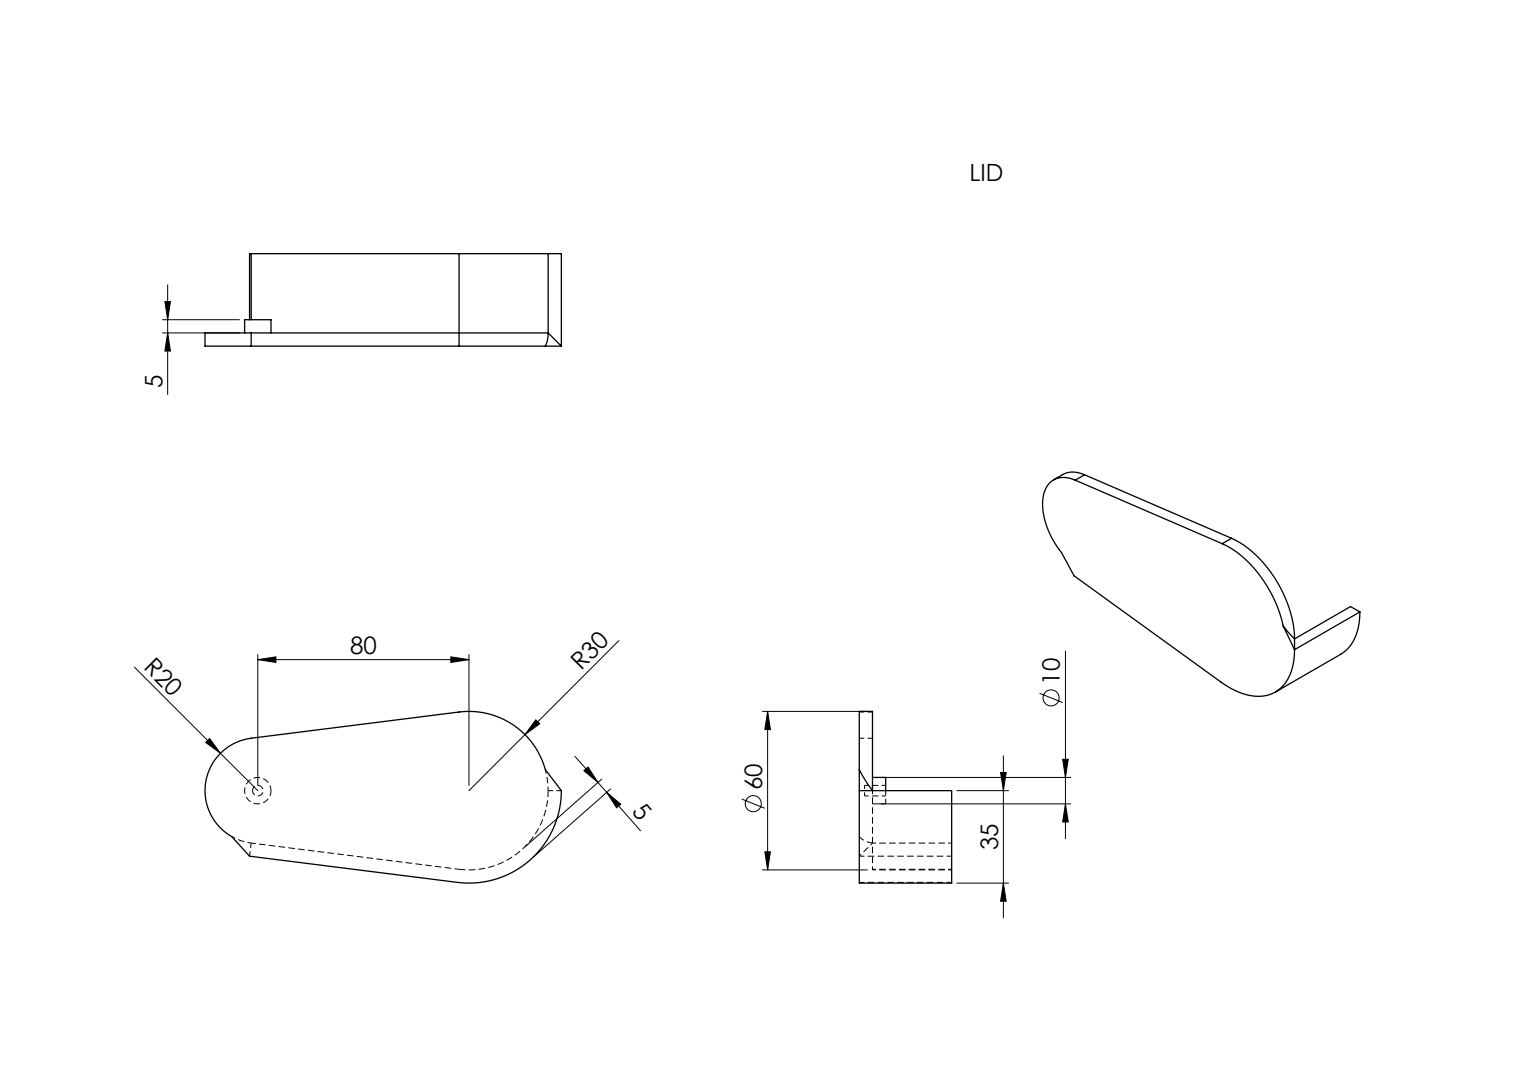
ISO-10303-21;
HEADER;
FILE_DESCRIPTION (('STEP AP214'),
    '1' );
FILE_NAME ('lid.step',
    '2026-10-24T08:20:21',
    ( '' ),
    ( '' ),
    'SwSTEP 2.0',
    'SolidWorks 2026',
    '' );
FILE_SCHEMA (( 'AUTOMOTIVE_DESIGN' ));
ENDSEC;

DATA;
#5=ORIENTED_EDGE ( 'NONE', *, *, #1076, .T. ) ;
#24=VECTOR ( 'NONE', #1964, 1000.000000000000000 ) ;
#27=CARTESIAN_POINT ( 'NONE',  ( -85.00000000000000000, 6.123233995736770227E-16, 0.000000000000000000 ) ) ;
#30=ORIENTED_EDGE ( 'NONE', *, *, #1022, .T. ) ;
#33=CIRCLE ( 'NONE', #906, 20.00000000000000355 ) ;
#34=EDGE_CURVE ( 'NONE', #3645, #1107, #2841, .T. ) ;
#40=COLOUR_RGB ( '',0.8941176470588234615, 0.8941176470588234615, 0.8941176470588234615 ) ;
#45=( LENGTH_UNIT ( ) NAMED_UNIT ( * ) SI_UNIT ( .MILLI., .METRE. ) );
#47=PLANE ( 'NONE',  #2813 ) ;
#66=CARTESIAN_POINT ( 'NONE',  ( -80.00000000000000000, 0.000000000000000000, -5.000000000000000000 ) ) ;
#68=CARTESIAN_POINT ( 'NONE',  ( -80.00000000000000000, 0.000000000000000000, 0.000000000000000000 ) ) ;
#73=CARTESIAN_POINT ( 'NONE',  ( -80.00000000000000000, 0.000000000000000000, -5.000000000000000000 ) ) ;
#86=ORIENTED_EDGE ( 'NONE', *, *, #1066, .F. ) ;
#92=CARTESIAN_POINT ( 'NONE',  ( 28.92857142857272379, 7.945926950454914817, 5.000000000000000000 ) ) ;
#100=EDGE_CURVE ( 'NONE', #2912, #2597, #2303, .T. ) ;
#119=DIRECTION ( 'NONE',  ( -0.000000000000000000, 0.000000000000000000, 1.000000000000000000 ) ) ;
#121=PLANE ( 'NONE',  #644 ) ;
#131=VECTOR ( 'NONE', #1399, 1000.000000000000000 ) ;
#132=AXIS2_PLACEMENT_3D ( 'NONE', #1292, #3708, #687 ) ;
#135=EDGE_LOOP ( 'NONE', ( #399, #815 ) ) ;
#138=CARTESIAN_POINT ( 'NONE',  ( -83.12500000000000000, -24.80391854123052653, 5.000000000000000000 ) ) ;
#145=EDGE_CURVE ( 'NONE', #3052, #3455, #33, .T. ) ;
#151=EDGE_CURVE ( 'NONE', #2912, #447, #915, .T. ) ;
#155=FACE_OUTER_BOUND ( 'NONE', #841, .T. ) ;
#157=EDGE_CURVE ( 'NONE', #2149, #2587, #627, .T. ) ;
#160=ORIENTED_EDGE ( 'NONE', *, *, #2560, .F. ) ;
#176=CARTESIAN_POINT ( 'NONE',  ( 0.000000000000000000, 0.000000000000000000, -30.00000000000000000 ) ) ;
#182=DIRECTION ( 'NONE',  ( -0.000000000000000000, 0.000000000000000000, 1.000000000000000000 ) ) ;
#183=ORIENTED_EDGE ( 'NONE', *, *, #151, .F. ) ;
#184=LINE ( 'NONE', #240, #851 ) ;
#187=CARTESIAN_POINT ( 'NONE',  ( -82.50000000000000000, -19.84313483298442904, 0.000000000000000000 ) ) ;
#194=FACE_OUTER_BOUND ( 'NONE', #457, .T. ) ;
#198=( GEOMETRIC_REPRESENTATION_CONTEXT ( 3 ) GLOBAL_UNCERTAINTY_ASSIGNED_CONTEXT ( ( #1403 ) ) GLOBAL_UNIT_ASSIGNED_CONTEXT ( ( #953, #339, #637 ) ) REPRESENTATION_CONTEXT ( 'NONE', 'WORKASPACE' ) );
#202=CARTESIAN_POINT ( 'NONE',  ( 28.92857142857272379, 7.945926950454914817, 5.000000000000000000 ) ) ;
#210=DIRECTION ( 'NONE',  ( 1.000000000000000000, 0.000000000000000000, 0.000000000000000000 ) ) ;
#217=CARTESIAN_POINT ( 'NONE',  ( -85.13135963406439544, -19.37413418176162594, 2.144658748104447454 ) ) ;
#222=FACE_OUTER_BOUND ( 'NONE', #2249, .T. ) ;
#228=CARTESIAN_POINT ( 'NONE',  ( -80.00000000000000000, 0.000000000000000000, -5.000000000000000000 ) ) ;
#230=EDGE_LOOP ( 'NONE', ( #423, #458, #2940, #857 ) ) ;
#236=B_SPLINE_CURVE_WITH_KNOTS ( 'NONE', 3,
 ( #2282, #3465, #1982, #3172 ),
 .UNSPECIFIED., .F., .F.,
 ( 4, 4 ),
 ( 0.000000000000000000, 1.000000000000000000 ),
 .UNSPECIFIED. ) ;
#238=PLANE ( 'NONE',  #1875 ) ;
#240=CARTESIAN_POINT ( 'NONE',  ( -4.374999999999999112, -34.72548595772274638, -30.00000000000000000 ) ) ;
#248=CARTESIAN_POINT ( 'NONE',  ( -4.375000000000000888, -34.72548595772274638, 5.000000000000000000 ) ) ;
#250=ADVANCED_FACE ( 'NONE', ( #2060 ), #299, .T. ) ;
#254=ORIENTED_EDGE ( 'NONE', *, *, #3594, .F. ) ;
#269=B_SPLINE_CURVE_WITH_KNOTS ( 'NONE', 3,
 ( #2225, #1680, #3784, #502 ),
 .UNSPECIFIED., .F., .F.,
 ( 4, 4 ),
 ( 0.000000000000000000, 1.000000000000000000 ),
 .UNSPECIFIED. ) ;
#272=VERTEX_POINT ( 'NONE', #897 ) ;
#288=B_SPLINE_CURVE_WITH_KNOTS ( 'NONE', 3,
 ( #1129, #864, #2961, #3833 ),
 .UNSPECIFIED., .F., .F.,
 ( 4, 4 ),
 ( 0.000000000000000000, 1.000000000000000000 ),
 .UNSPECIFIED. ) ;
#292=DIRECTION ( 'NONE',  ( 0.000000000000000000, 0.000000000000000000, 1.000000000000000000 ) ) ;
#297=ORIENTED_EDGE ( 'NONE', *, *, #1259, .F. ) ;
#299=CYLINDRICAL_SURFACE ( 'NONE', #1463, 20.00000000000000355 ) ;
#305=DIRECTION ( 'NONE',  ( -0.9921567416492215186, 0.1250000000000000833, 0.000000000000000000 ) ) ;
#318=VECTOR ( 'NONE', #1119, 999.9999999999998863 ) ;
#323=VECTOR ( 'NONE', #1438, 1000.000000000000114 ) ;
#327=AXIS2_PLACEMENT_3D ( 'NONE', #856, #2331, #1108 ) ;
#329=PLANE ( 'NONE',  #132 ) ;
#339=( NAMED_UNIT ( * ) PLANE_ANGLE_UNIT ( ) SI_UNIT ( $, .RADIAN. ) );
#340=MECHANICAL_DESIGN_GEOMETRIC_PRESENTATION_REPRESENTATION('',(#468),#3515);
#343=PRODUCT ( 'lid', 'lid', '', ( #1165 ) ) ;
#356=LINE ( 'NONE', #1470, #3071 ) ;
#371=CARTESIAN_POINT ( 'NONE',  ( 34.99999999999999289, 0.000000000000000000, -30.00000000000000000 ) ) ;
#382=EDGE_CURVE ( 'NONE', #2840, #3645, #603, .T. ) ;
#388=EDGE_CURVE ( 'NONE', #973, #1542, #2135, .T. ) ;
#392=CARTESIAN_POINT ( 'NONE',  ( 30.00000000000000000, 0.000000000000000000, -15.00000000000000000 ) ) ;
#399=ORIENTED_EDGE ( 'NONE', *, *, #1610, .T. ) ;
#403=VECTOR ( 'NONE', #2056, 1000.000000000000000 ) ;
#405=DIRECTION ( 'NONE',  ( 0.000000000000000000, 0.000000000000000000, 1.000000000000000000 ) ) ;
#407=FACE_OUTER_BOUND ( 'NONE', #796, .T. ) ;
#414=LINE ( 'NONE', #2795, #24 ) ;
#415=EDGE_LOOP ( 'NONE', ( #3354, #1082 ) ) ;
#422=EDGE_CURVE ( 'NONE', #2840, #2012, #3114, .T. ) ;
#423=ORIENTED_EDGE ( 'NONE', *, *, #3594, .T. ) ;
#430=CARTESIAN_POINT ( 'NONE',  ( 0.000000000000000000, 0.000000000000000000, -30.00000000000000000 ) ) ;
#447=VERTEX_POINT ( 'NONE', #1262 ) ;
#453=EDGE_LOOP ( 'NONE', ( #297, #1815, #2065, #876 ) ) ;
#456=FACE_OUTER_BOUND ( 'NONE', #836, .T. ) ;
#457=EDGE_LOOP ( 'NONE', ( #3256, #3221, #3322, #30 ) ) ;
#458=ORIENTED_EDGE ( 'NONE', *, *, #1532, .F. ) ;
#468=STYLED_ITEM ( 'NONE', ( #939 ), #3116 ) ;
#490=LINE ( 'NONE', #3484, #318 ) ;
#502=CARTESIAN_POINT ( 'NONE',  ( 28.92857142857272379, 7.945926950454914817, 5.000000000000000000 ) ) ;
#503=ORIENTED_EDGE ( 'NONE', *, *, #2320, .F. ) ;
#505=CARTESIAN_POINT ( 'NONE',  ( -82.50000000000000000, -19.84313483298442904, 0.000000000000000000 ) ) ;
#506=EDGE_LOOP ( 'NONE', ( #2013, #1714, #3610, #3275 ) ) ;
#534=DIRECTION ( 'NONE',  ( 0.6221102074731698073, 0.4753501651576230724, -0.6221102074731695852 ) ) ;
#536=CARTESIAN_POINT ( 'NONE',  ( -4.375000000000001776, -34.72548595772274638, -30.00000000000000000 ) ) ;
#537=PRODUCT_DEFINITION ( 'UNKNOWN', '', #3334, #2544 ) ;
#541=DIRECTION ( 'NONE',  ( -0.000000000000000000, -0.000000000000000000, 1.000000000000000000 ) ) ;
#571=ORIENTED_EDGE ( 'NONE', *, *, #2102, .F. ) ;
#577=AXIS2_PLACEMENT_3D ( 'NONE', #710, #3339, #1868 ) ;
#603=LINE ( 'NONE', #2116, #3452 ) ;
#613=ORIENTED_EDGE ( 'NONE', *, *, #1657, .T. ) ;
#627=B_SPLINE_CURVE_WITH_KNOTS ( 'NONE', 3,
 ( #187, #1692, #2876, #2337 ),
 .UNSPECIFIED., .F., .F.,
 ( 4, 4 ),
 ( 0.000000000000000000, 1.000000000000000000 ),
 .UNSPECIFIED. ) ;
#633=ORIENTED_EDGE ( 'NONE', *, *, #1532, .T. ) ;
#637=( NAMED_UNIT ( * ) SI_UNIT ( $, .STERADIAN. ) SOLID_ANGLE_UNIT ( ) );
#642=CARTESIAN_POINT ( 'NONE',  ( 29.64285714285758999, 5.345441766669614125, 3.727272727272256336 ) ) ;
#644=AXIS2_PLACEMENT_3D ( 'NONE', #2215, #2193, #3654 ) ;
#645=AXIS2_PLACEMENT_3D ( 'NONE', #68, #3596, #933 ) ;
#651=ORIENTED_EDGE ( 'NONE', *, *, #3049, .T. ) ;
#658=LINE ( 'NONE', #1244, #2009 ) ;
#663=( NAMED_UNIT ( * ) SI_UNIT ( $, .STERADIAN. ) SOLID_ANGLE_UNIT ( ) );
#664=AXIS2_PLACEMENT_3D ( 'NONE', #2506, #2533, #3696 ) ;
#670=DIRECTION ( 'NONE',  ( -0.1250000000000000555, -0.9921567416492214075, 0.000000000000000000 ) ) ;
#680=( LENGTH_UNIT ( ) NAMED_UNIT ( * ) SI_UNIT ( .MILLI., .METRE. ) );
#687=DIRECTION ( 'NONE',  ( -1.000000000000000000, 0.000000000000000000, -0.000000000000000000 ) ) ;
#700=SHAPE_REPRESENTATION_RELATIONSHIP ( 'NONE' , 'NONE' ,  #2152, #3116 ) ;
#704=AXIS2_PLACEMENT_3D ( 'NONE', #430, #1338, #1604 ) ;
#706=CARTESIAN_POINT ( 'NONE',  ( -3.749999999999998224, -29.76470224947664533, 0.000000000000000000 ) ) ;
#709=ORIENTED_EDGE ( 'NONE', *, *, #3416, .F. ) ;
#710=CARTESIAN_POINT ( 'NONE',  ( -78.00000000000000000, 0.000000000000000000, 3.000000000000000000 ) ) ;
#720=AXIS2_PLACEMENT_3D ( 'NONE', #176, #788, #1721 ) ;
#722=DIRECTION ( 'NONE',  ( 1.000000000000000000, 0.000000000000000000, 0.000000000000000000 ) ) ;
#733=DIRECTION ( 'NONE',  ( -1.000000000000000000, 0.000000000000000000, 0.000000000000000000 ) ) ;
#734=EDGE_CURVE ( 'NONE', #916, #926, #1606, .T. ) ;
#735=DIRECTION ( 'NONE',  ( 1.000000000000000000, 0.000000000000000000, 0.000000000000000000 ) ) ;
#743=CARTESIAN_POINT ( 'NONE',  ( -80.00000000000000000, 0.000000000000000000, -5.000000000000000000 ) ) ;
#752=DIRECTION ( 'NONE',  ( 0.9921567416492214075, 0.1250000000000001388, 0.000000000000000000 ) ) ;
#753=ORIENTED_EDGE ( 'NONE', *, *, #1610, .F. ) ;
#754=CARTESIAN_POINT ( 'NONE',  ( 34.99999999999999289, 0.000000000000000000, 4.999999999999997335 ) ) ;
#756=FACE_OUTER_BOUND ( 'NONE', #3199, .T. ) ;
#763=CIRCLE ( 'NONE', #1018, 34.99999999999999289 ) ;
#765=CIRCLE ( 'NONE', #2944, 2.000000000000001776 ) ;
#773=ORIENTED_EDGE ( 'NONE', *, *, #2847, .T. ) ;
#780=CARTESIAN_POINT ( 'NONE',  ( -82.50000000000000000, 19.84313483298442193, 0.000000000000000000 ) ) ;
#788=DIRECTION ( 'NONE',  ( 0.000000000000000000, 0.000000000000000000, 1.000000000000000000 ) ) ;
#796=EDGE_LOOP ( 'NONE', ( #3689, #2096 ) ) ;
#806=DIRECTION ( 'NONE',  ( -0.9921567416492214075, 0.1250000000000000555, 0.000000000000000000 ) ) ;
#815=ORIENTED_EDGE ( 'NONE', *, *, #2560, .T. ) ;
#819=DIRECTION ( 'NONE',  ( 0.000000000000000000, 0.000000000000000000, 1.000000000000000000 ) ) ;
#820=CARTESIAN_POINT ( 'NONE',  ( 0.000000000000000000, 0.000000000000000000, 0.000000000000000000 ) ) ;
#821=VERTEX_POINT ( 'NONE', #3348 ) ;
#822=VECTOR ( 'NONE', #1593, 999.9999999999998863 ) ;
#828=UNCERTAINTY_MEASURE_WITH_UNIT (LENGTH_MEASURE( 1.000000000000000082E-05 ), #45, 'distance_accuracy_value', 'NONE');
#831=FACE_OUTER_BOUND ( 'NONE', #3651, .T. ) ;
#832=VECTOR ( 'NONE', #405, 1000.000000000000000 ) ;
#836=EDGE_LOOP ( 'NONE', ( #1395, #5, #966, #3713, #3401, #3386 ) ) ;
#837=CARTESIAN_POINT ( 'NONE',  ( -80.00000000000000000, 0.000000000000000000, 5.000000000000000000 ) ) ;
#841=EDGE_LOOP ( 'NONE', ( #254, #990, #1674, #1273, #1658, #1329, #1704 ) ) ;
#845=ADVANCED_FACE ( 'NONE', ( #3670 ), #1013, .T. ) ;
#851=VECTOR ( 'NONE', #3438, 1000.000000000000000 ) ;
#856=CARTESIAN_POINT ( 'NONE',  ( 0.000000000000000000, 0.000000000000000000, 0.000000000000000000 ) ) ;
#857=ORIENTED_EDGE ( 'NONE', *, *, #1052, .T. ) ;
#860=ADVANCED_FACE ( 'NONE', ( #1357 ), #1602, .T. ) ;
#864=CARTESIAN_POINT ( 'NONE',  ( -85.36741282452705093, -22.33760634779116572, 4.999999999999999112 ) ) ;
#868=VERTEX_POINT ( 'NONE', #2547 ) ;
#869=LINE ( 'NONE', #2673, #2691 ) ;
#876=ORIENTED_EDGE ( 'NONE', *, *, #1758, .T. ) ;
#879=ORIENTED_EDGE ( 'NONE', *, *, #3782, .F. ) ;
#882=ORIENTED_EDGE ( 'NONE', *, *, #3649, .T. ) ;
#893=MECHANICAL_DESIGN_GEOMETRIC_PRESENTATION_REPRESENTATION('',(#2124),#198);
#897=CARTESIAN_POINT ( 'NONE',  ( -82.00000000000000000, 0.000000000000000000, 3.000000000000000000 ) ) ;
#906=AXIS2_PLACEMENT_3D ( 'NONE', #837, #3174, #2024 ) ;
#910=VERTEX_POINT ( 'NONE', #1069 ) ;
#913=AXIS2_PLACEMENT_3D ( 'NONE', #1710, #2640, #3753 ) ;
#915=CIRCLE ( 'NONE', #2590, 5.000000000000004441 ) ;
#916=VERTEX_POINT ( 'NONE', #371 ) ;
#926=VERTEX_POINT ( 'NONE', #754 ) ;
#930=EDGE_CURVE ( 'NONE', #1166, #1798, #1457, .T. ) ;
#933=DIRECTION ( 'NONE',  ( 1.000000000000000000, 0.000000000000000000, 0.000000000000000000 ) ) ;
#939=PRESENTATION_STYLE_ASSIGNMENT (( #2140 ) ) ;
#941=CARTESIAN_POINT ( 'NONE',  ( -82.50000000000000000, -19.84313483298442904, -30.00000000000000000 ) ) ;
#951=DIRECTION ( 'NONE',  ( 0.000000000000000000, 0.000000000000000000, 1.000000000000000000 ) ) ;
#953=( LENGTH_UNIT ( ) NAMED_UNIT ( * ) SI_UNIT ( .MILLI., .METRE. ) );
#965=FACE_BOUND ( 'NONE', #415, .T. ) ;
#966=ORIENTED_EDGE ( 'NONE', *, *, #3281, .F. ) ;
#973=VERTEX_POINT ( 'NONE', #3419 ) ;
#974=CARTESIAN_POINT ( 'NONE',  ( -3.749999999999998224, -29.76470224947664533, -30.00000000000000000 ) ) ;
#980=FILL_AREA_STYLE_COLOUR ( '', #40 ) ;
#987=CARTESIAN_POINT ( 'NONE',  ( -3.750000000000001776, -29.76470224947664178, 0.000000000000000000 ) ) ;
#988=B_SPLINE_CURVE_WITH_KNOTS ( 'NONE', 3,
 ( #1809, #2416, #642, #92 ),
 .UNSPECIFIED., .F., .F.,
 ( 4, 4 ),
 ( 0.000000000000000000, 1.000000000000000000 ),
 .UNSPECIFIED. ) ;
#990=ORIENTED_EDGE ( 'NONE', *, *, #1849, .T. ) ;
#1004=DIRECTION ( 'NONE',  ( -0.000000000000000000, -0.000000000000000000, -1.000000000000000000 ) ) ;
#1005=PRODUCT_DEFINITION_SHAPE ( 'NONE', 'NONE',  #537 ) ;
#1013=CYLINDRICAL_SURFACE ( 'NONE', #1035, 34.99999999999999289 ) ;
#1015=CARTESIAN_POINT ( 'NONE',  ( 0.000000000000000000, 0.000000000000000000, 4.999999999999997335 ) ) ;
#1018=AXIS2_PLACEMENT_3D ( 'NONE', #1015, #3387, #2507 ) ;
#1022=EDGE_CURVE ( 'NONE', #2012, #2149, #2017, .T. ) ;
#1028=CARTESIAN_POINT ( 'NONE',  ( -80.00000000000000000, 0.000000000000000000, -5.000000000000000000 ) ) ;
#1035=AXIS2_PLACEMENT_3D ( 'NONE', #2174, #3363, #722 ) ;
#1038=CARTESIAN_POINT ( 'NONE',  ( -3.750000000000004441, 29.76470224947664533, 5.000000000000000000 ) ) ;
#1042=ADVANCED_FACE ( 'NONE', ( #2538 ), #3161, .F. ) ;
#1048=ORIENTED_EDGE ( 'NONE', *, *, #1638, .T. ) ;
#1050=FACE_OUTER_BOUND ( 'NONE', #2059, .T. ) ;
#1052=EDGE_CURVE ( 'NONE', #868, #3489, #184, .T. ) ;
#1060=FACE_OUTER_BOUND ( 'NONE', #3394, .T. ) ;
#1066=EDGE_CURVE ( 'NONE', #2840, #2084, #3460, .T. ) ;
#1069=CARTESIAN_POINT ( 'NONE',  ( -3.749999999999998224, 29.76470224947664533, 0.000000000000000000 ) ) ;
#1071=CARTESIAN_POINT ( 'NONE',  ( 30.00000000000000000, 0.000000000000000000, -30.00000000000000000 ) ) ;
#1074=DIRECTION ( 'NONE',  ( 0.000000000000000000, 0.000000000000000000, -1.000000000000000000 ) ) ;
#1076=EDGE_CURVE ( 'NONE', #868, #821, #3171, .T. ) ;
#1079=DIRECTION ( 'NONE',  ( 1.000000000000000000, 0.000000000000000000, 0.000000000000000000 ) ) ;
#1082=ORIENTED_EDGE ( 'NONE', *, *, #2401, .F. ) ;
#1083=DIRECTION ( 'NONE',  ( 0.1250000000000000833, 0.9921567416492215186, -0.000000000000000000 ) ) ;
#1100=EDGE_CURVE ( 'NONE', #1755, #2149, #3706, .T. ) ;
#1106=FACE_OUTER_BOUND ( 'NONE', #230, .T. ) ;
#1107=VERTEX_POINT ( 'NONE', #1999 ) ;
#1108=DIRECTION ( 'NONE',  ( 1.000000000000000000, 0.000000000000000000, 0.000000000000000000 ) ) ;
#1116=CARTESIAN_POINT ( 'NONE',  ( -78.00000000000000000, 2.449293598294708880E-16, -5.000000000000000000 ) ) ;
#1119=DIRECTION ( 'NONE',  ( 0.9921567416492215186, 0.1250000000000001665, 0.000000000000000000 ) ) ;
#1128=CARTESIAN_POINT ( 'NONE',  ( -80.00000000000000000, 0.000000000000000000, -5.000000000000000000 ) ) ;
#1129=CARTESIAN_POINT ( 'NONE',  ( -83.12500000000000000, -24.80391854123052653, 5.000000000000000000 ) ) ;
#1135=CARTESIAN_POINT ( 'NONE',  ( -87.59475001958765006, -18.54744454438354495, 3.811325414771110864 ) ) ;
#1141=FACE_OUTER_BOUND ( 'NONE', #1390, .T. ) ;
#1157=ORIENTED_EDGE ( 'NONE', *, *, #34, .T. ) ;
#1165=PRODUCT_CONTEXT ( 'NONE', #3024, 'mechanical' ) ;
#1166=VERTEX_POINT ( 'NONE', #202 ) ;
#1167=DIRECTION ( 'NONE',  ( -0.000000000000000000, -0.000000000000000000, -1.000000000000000000 ) ) ;
#1179=CARTESIAN_POINT ( 'NONE',  ( -3.749999999999998224, 29.76470224947664533, 0.000000000000000000 ) ) ;
#1180=ADVANCED_FACE ( 'NONE', ( #831 ), #2473, .F. ) ;
#1221=VECTOR ( 'NONE', #1981, 1000.000000000000114 ) ;
#1231=DIRECTION ( 'NONE',  ( -1.000000000000000000, 0.000000000000000000, 0.000000000000000000 ) ) ;
#1244=CARTESIAN_POINT ( 'NONE',  ( -82.50000000000000000, 19.84313483298442193, 0.000000000000000000 ) ) ;
#1259=EDGE_CURVE ( 'NONE', #910, #1798, #3531, .T. ) ;
#1262=CARTESIAN_POINT ( 'NONE',  ( -85.00000000000000000, 6.123233995736770227E-16, -5.000000000000000000 ) ) ;
#1273=ORIENTED_EDGE ( 'NONE', *, *, #930, .T. ) ;
#1276=CARTESIAN_POINT ( 'NONE',  ( -80.00000000000000000, 0.000000000000000000, 3.000000000000000000 ) ) ;
#1279=AXIS2_PLACEMENT_3D ( 'NONE', #3641, #2163, #1885 ) ;
#1285=VECTOR ( 'NONE', #3099, 999.9999999999998863 ) ;
#1292=CARTESIAN_POINT ( 'NONE',  ( -80.00000000000000000, 0.000000000000000000, -5.000000000000000000 ) ) ;
#1305=FACE_OUTER_BOUND ( 'NONE', #2952, .T. ) ;
#1313=CARTESIAN_POINT ( 'NONE',  ( 0.000000000000000000, 0.000000000000000000, 5.000000000000000000 ) ) ;
#1315=CIRCLE ( 'NONE', #2746, 2.000000000000001776 ) ;
#1321=AXIS2_PLACEMENT_3D ( 'NONE', #228, #541, #210 ) ;
#1329=ORIENTED_EDGE ( 'NONE', *, *, #145, .T. ) ;
#1333=ORIENTED_EDGE ( 'NONE', *, *, #3449, .T. ) ;
#1338=DIRECTION ( 'NONE',  ( 0.000000000000000000, 0.000000000000000000, -1.000000000000000000 ) ) ;
#1343=DIRECTION ( 'NONE',  ( -1.000000000000000000, 0.000000000000000000, 0.000000000000000000 ) ) ;
#1357=FACE_OUTER_BOUND ( 'NONE', #2852, .T. ) ;
#1361=ORIENTED_EDGE ( 'NONE', *, *, #388, .T. ) ;
#1362=DIRECTION ( 'NONE',  ( -1.000000000000000000, 0.000000000000000000, 0.000000000000000000 ) ) ;
#1373=CARTESIAN_POINT ( 'NONE',  ( -82.50000000000000000, 19.84313483298442193, 5.000000000000000000 ) ) ;
#1384=AXIS2_PLACEMENT_3D ( 'NONE', #3193, #1720, #2904 ) ;
#1390=EDGE_LOOP ( 'NONE', ( #2719, #2420, #1333, #2005, #1429 ) ) ;
#1395=ORIENTED_EDGE ( 'NONE', *, *, #1571, .F. ) ;
#1399=DIRECTION ( 'NONE',  ( -0.000000000000000000, -0.000000000000000000, 1.000000000000000000 ) ) ;
#1403=UNCERTAINTY_MEASURE_WITH_UNIT (LENGTH_MEASURE( 1.000000000000000082E-05 ), #953, 'distance_accuracy_value', 'NONE');
#1415=ORIENTED_EDGE ( 'NONE', *, *, #2974, .T. ) ;
#1417=CYLINDRICAL_SURFACE ( 'NONE', #1321, 5.000000000000004441 ) ;
#1419=ADVANCED_FACE ( 'NONE', ( #1305 ), #2489, .T. ) ;
#1425=DIRECTION ( 'NONE',  ( 0.3361233252211006661, -0.8797966926992965009, -0.3361233252211005551 ) ) ;
#1429=ORIENTED_EDGE ( 'NONE', *, *, #34, .F. ) ;
#1438=DIRECTION ( 'NONE',  ( -0.9921567416492214075, 0.1250000000000000555, 0.000000000000000000 ) ) ;
#1450=ORIENTED_EDGE ( 'NONE', *, *, #1259, .T. ) ;
#1457=CIRCLE ( 'NONE', #3637, 30.00000000000000000 ) ;
#1458=ADVANCED_FACE ( 'NONE', ( #155 ), #3142, .T. ) ;
#1463=AXIS2_PLACEMENT_3D ( 'NONE', #3018, #3597, #1803 ) ;
#1468=DIRECTION ( 'NONE',  ( -0.000000000000000000, -0.000000000000000000, -1.000000000000000000 ) ) ;
#1470=CARTESIAN_POINT ( 'NONE',  ( -82.00000000000000000, 0.000000000000000000, -5.000000000000000000 ) ) ;
#1480=EDGE_CURVE ( 'NONE', #447, #2912, #2805, .T. ) ;
#1511=CIRCLE ( 'NONE', #1953, 30.00000000000000000 ) ;
#1512=DIRECTION ( 'NONE',  ( -0.000000000000000000, -0.000000000000000000, -1.000000000000000000 ) ) ;
#1529=DIRECTION ( 'NONE',  ( -0.000000000000000000, -0.000000000000000000, -1.000000000000000000 ) ) ;
#1532=EDGE_CURVE ( 'NONE', #821, #2587, #869, .T. ) ;
#1542=VERTEX_POINT ( 'NONE', #1116 ) ;
#1560=CARTESIAN_POINT ( 'NONE',  ( -3.750000000000004441, 29.76470224947664533, 0.000000000000000000 ) ) ;
#1561=ORIENTED_EDGE ( 'NONE', *, *, #2401, .T. ) ;
#1567=VECTOR ( 'NONE', #670, 1000.000000000000114 ) ;
#1571=EDGE_CURVE ( 'NONE', #868, #916, #3242, .T. ) ;
#1574=CARTESIAN_POINT ( 'NONE',  ( 30.00000000000000000, 0.000000000000000000, -30.00000000000000000 ) ) ;
#1584=AXIS2_PLACEMENT_3D ( 'NONE', #3222, #2581, #3154 ) ;
#1593=DIRECTION ( 'NONE',  ( 0.9921567416492215186, 0.1250000000000001665, 0.000000000000000000 ) ) ;
#1602=PLANE ( 'NONE',  #3454 ) ;
#1604=DIRECTION ( 'NONE',  ( -1.000000000000000000, 0.000000000000000000, -0.000000000000000000 ) ) ;
#1606=LINE ( 'NONE', #1922, #3206 ) ;
#1610=EDGE_CURVE ( 'NONE', #272, #973, #2433, .T. ) ;
#1614=VERTEX_POINT ( 'NONE', #3061 ) ;
#1638=EDGE_CURVE ( 'NONE', #1107, #1166, #988, .T. ) ;
#1640=CARTESIAN_POINT ( 'NONE',  ( -89.85223847358115279, -17.40498196091244409, 5.000000000000000000 ) ) ;
#1643=UNCERTAINTY_MEASURE_WITH_UNIT (LENGTH_MEASURE( 1.000000000000000082E-05 ), #680, 'distance_accuracy_value', 'NONE');
#1655=CARTESIAN_POINT ( 'NONE',  ( -3.749999999999998224, 29.76470224947664533, 5.000000000000000000 ) ) ;
#1657=EDGE_CURVE ( 'NONE', #1614, #1542, #1315, .T. ) ;
#1658=ORIENTED_EDGE ( 'NONE', *, *, #1758, .F. ) ;
#1660=CARTESIAN_POINT ( 'NONE',  ( 0.000000000000000000, 0.000000000000000000, 5.000000000000000000 ) ) ;
#1664=EDGE_LOOP ( 'NONE', ( #3316, #2404, #2850, #633 ) ) ;
#1674=ORIENTED_EDGE ( 'NONE', *, *, #3782, .T. ) ;
#1680=CARTESIAN_POINT ( 'NONE',  ( 32.97619047619090793, 2.648642316818304643, 5.000000000000000000 ) ) ;
#1692=CARTESIAN_POINT ( 'NONE',  ( -82.70833333333334281, -21.49672940239979724, 1.666666666666666297 ) ) ;
#1704=ORIENTED_EDGE ( 'NONE', *, *, #1939, .F. ) ;
#1710=CARTESIAN_POINT ( 'NONE',  ( 0.000000000000000000, 0.000000000000000000, -30.00000000000000000 ) ) ;
#1714=ORIENTED_EDGE ( 'NONE', *, *, #734, .T. ) ;
#1720=DIRECTION ( 'NONE',  ( 0.000000000000000000, 0.000000000000000000, 1.000000000000000000 ) ) ;
#1721=DIRECTION ( 'NONE',  ( 1.000000000000000000, 0.000000000000000000, 0.000000000000000000 ) ) ;
#1725=B_SPLINE_CURVE_WITH_KNOTS ( 'NONE', 3,
 ( #505, #3456, #217, #1135, #3786, #1640 ),
 .UNSPECIFIED., .F., .F.,
 ( 4, 2, 4 ),
 ( 0.000000000000000000, 0.5000000000000000000, 1.000000000000000000 ),
 .UNSPECIFIED. ) ;
#1727=DIRECTION ( 'NONE',  ( 0.000000000000000000, 0.000000000000000000, 1.000000000000000000 ) ) ;
#1755=VERTEX_POINT ( 'NONE', #780 ) ;
#1756=AXIS2_PLACEMENT_3D ( 'NONE', #2851, #1083, #2557 ) ;
#1758=EDGE_CURVE ( 'NONE', #3052, #1798, #3758, .T. ) ;
#1759=EDGE_LOOP ( 'NONE', ( #2666, #2127 ) ) ;
#1763=AXIS2_PLACEMENT_3D ( 'NONE', #1276, #1004, #733 ) ;
#1778=VECTOR ( 'NONE', #1727, 1000.000000000000000 ) ;
#1796=FACE_OUTER_BOUND ( 'NONE', #1664, .T. ) ;
#1798=VERTEX_POINT ( 'NONE', #1655 ) ;
#1803=DIRECTION ( 'NONE',  ( 1.000000000000000000, 0.000000000000000000, 0.000000000000000000 ) ) ;
#1809=CARTESIAN_POINT ( 'NONE',  ( 30.00000000000000000, 0.000000000000000000, 0.000000000000000000 ) ) ;
#1815=ORIENTED_EDGE ( 'NONE', *, *, #3449, .F. ) ;
#1849=EDGE_CURVE ( 'NONE', #3489, #926, #763, .T. ) ;
#1856=FACE_OUTER_BOUND ( 'NONE', #453, .T. ) ;
#1859=ADVANCED_FACE ( 'NONE', ( #2221 ), #3407, .F. ) ;
#1860=CARTESIAN_POINT ( 'NONE',  ( -3.750000000000001776, -29.76470224947664178, -30.00000000000000000 ) ) ;
#1866=ADVANCED_FACE ( 'NONE', ( #1060 ), #1417, .T. ) ;
#1868=DIRECTION ( 'NONE',  ( 1.000000000000000000, 0.000000000000000000, -0.000000000000000000 ) ) ;
#1875=AXIS2_PLACEMENT_3D ( 'NONE', #1997, #534, #1425 ) ;
#1883=CIRCLE ( 'NONE', #645, 5.000000000000004441 ) ;
#1885=DIRECTION ( 'NONE',  ( -1.000000000000000000, 0.000000000000000000, 0.000000000000000000 ) ) ;
#1900=CARTESIAN_POINT ( 'NONE',  ( -75.00000000000000000, 0.000000000000000000, -5.000000000000000000 ) ) ;
#1922=CARTESIAN_POINT ( 'NONE',  ( 34.99999999999999289, 0.000000000000000000, -30.00000000000000000 ) ) ;
#1923=ORIENTED_EDGE ( 'NONE', *, *, #1100, .T. ) ;
#1924=DIRECTION ( 'NONE',  ( -0.000000000000000000, -0.000000000000000000, -1.000000000000000000 ) ) ;
#1937=CARTESIAN_POINT ( 'NONE',  ( -82.50000000000000000, -19.84313483298442904, 0.000000000000000000 ) ) ;
#1939=EDGE_CURVE ( 'NONE', #2587, #3455, #288, .T. ) ;
#1953=AXIS2_PLACEMENT_3D ( 'NONE', #2599, #182, #2298 ) ;
#1964=DIRECTION ( 'NONE',  ( 1.000000000000000000, 0.000000000000000000, 0.000000000000000000 ) ) ;
#1981=DIRECTION ( 'NONE',  ( -0.9921567416492214075, 0.1250000000000000555, 0.000000000000000000 ) ) ;
#1982=CARTESIAN_POINT ( 'NONE',  ( 33.33333333333333570, 0.000000000000000000, 3.333333333333331705 ) ) ;
#1983=EDGE_CURVE ( 'NONE', #1755, #3052, #658, .T. ) ;
#1991=EDGE_LOOP ( 'NONE', ( #160, #1361, #1561, #2928 ) ) ;
#1997=CARTESIAN_POINT ( 'NONE',  ( 34.99999999999999289, 0.000000000000000000, 5.000000000000000000 ) ) ;
#1999=CARTESIAN_POINT ( 'NONE',  ( 30.00000000000000000, 0.000000000000000000, 0.000000000000000000 ) ) ;
#2005=ORIENTED_EDGE ( 'NONE', *, *, #3049, .F. ) ;
#2009=VECTOR ( 'NONE', #2136, 1000.000000000000000 ) ;
#2012=VERTEX_POINT ( 'NONE', #3554 ) ;
#2013=ORIENTED_EDGE ( 'NONE', *, *, #1571, .T. ) ;
#2014=CIRCLE ( 'NONE', #2761, 5.000000000000004441 ) ;
#2017=LINE ( 'NONE', #2893, #1778 ) ;
#2021=MANIFOLD_SOLID_BREP ( 'AdvancedHole1', #2664 ) ;
#2024=DIRECTION ( 'NONE',  ( 1.000000000000000000, 0.000000000000000000, 0.000000000000000000 ) ) ;
#2042=ADVANCED_FACE ( 'NONE', ( #756 ), #121, .T. ) ;
#2056=DIRECTION ( 'NONE',  ( -0.000000000000000000, 0.000000000000000000, 1.000000000000000000 ) ) ;
#2059=EDGE_LOOP ( 'NONE', ( #2408, #183, #3661, #1415 ) ) ;
#2060=FACE_OUTER_BOUND ( 'NONE', #2676, .T. ) ;
#2065=ORIENTED_EDGE ( 'NONE', *, *, #1983, .T. ) ;
#2084=VERTEX_POINT ( 'NONE', #1071 ) ;
#2096=ORIENTED_EDGE ( 'NONE', *, *, #1480, .T. ) ;
#2098=ADVANCED_FACE ( 'NONE', ( #456 ), #3076, .T. ) ;
#2102=EDGE_CURVE ( 'NONE', #2084, #916, #414, .T. ) ;
#2116=CARTESIAN_POINT ( 'NONE',  ( -3.749999999999998224, -29.76470224947664533, -30.00000000000000000 ) ) ;
#2124=STYLED_ITEM('',(#3860),#2021);
#2127=ORIENTED_EDGE ( 'NONE', *, *, #2821, .F. ) ;
#2135=LINE ( 'NONE', #3324, #3151 ) ;
#2136=DIRECTION ( 'NONE',  ( -0.000000000000000000, 0.000000000000000000, 1.000000000000000000 ) ) ;
#2140=SURFACE_STYLE_USAGE ( .BOTH. , #3044 ) ;
#2148=PLANE ( 'NONE',  #577 ) ;
#2149=VERTEX_POINT ( 'NONE', #1937 ) ;
#2152=SHAPE_REPRESENTATION ( 'lid', ( #2207 ), #3459 ) ;
#2156=DIRECTION ( 'NONE',  ( -0.000000000000000000, -0.000000000000000000, 1.000000000000000000 ) ) ;
#2160=DIRECTION ( 'NONE',  ( 0.000000000000000000, 0.000000000000000000, 1.000000000000000000 ) ) ;
#2162=( NAMED_UNIT ( * ) PLANE_ANGLE_UNIT ( ) SI_UNIT ( $, .RADIAN. ) );
#2163=DIRECTION ( 'NONE',  ( -0.000000000000000000, -0.000000000000000000, -1.000000000000000000 ) ) ;
#2167=CYLINDRICAL_SURFACE ( 'NONE', #2822, 5.000000000000004441 ) ;
#2174=CARTESIAN_POINT ( 'NONE',  ( 0.000000000000000000, 0.000000000000000000, -30.00000000000000000 ) ) ;
#2185=LINE ( 'NONE', #987, #2266 ) ;
#2193=DIRECTION ( 'NONE',  ( -0.5890940290687334269, -0.5356142702249980792, -0.6050500627608503823 ) ) ;
#2198=FILL_AREA_STYLE ('',( #980 ) ) ;
#2207=AXIS2_PLACEMENT_3D ( 'NONE', #820, #2246, #3194 ) ;
#2211=CARTESIAN_POINT ( 'NONE',  ( -80.00000000000000000, 0.000000000000000000, 0.000000000000000000 ) ) ;
#2212=ORIENTED_EDGE ( 'NONE', *, *, #157, .T. ) ;
#2215=CARTESIAN_POINT ( 'NONE',  ( -89.85223847358115279, -17.40498196091244409, 5.000000000000000000 ) ) ;
#2221=FACE_OUTER_BOUND ( 'NONE', #1991, .T. ) ;
#2225=CARTESIAN_POINT ( 'NONE',  ( 34.99999999999999289, 0.000000000000000000, 4.999999999999997335 ) ) ;
#2229=DIRECTION ( 'NONE',  ( 1.000000000000000000, 0.000000000000000000, 0.000000000000000000 ) ) ;
#2244=SHAPE_DEFINITION_REPRESENTATION ( #1005, #2152 ) ;
#2246=DIRECTION ( 'NONE',  ( 0.000000000000000000, 0.000000000000000000, 1.000000000000000000 ) ) ;
#2249=EDGE_LOOP ( 'NONE', ( #503, #1048, #879 ) ) ;
#2266=VECTOR ( 'NONE', #2774, 999.9999999999998863 ) ;
#2271=DIRECTION ( 'NONE',  ( 0.1250000000000000833, 0.9921567416492215186, -0.000000000000000000 ) ) ;
#2282=CARTESIAN_POINT ( 'NONE',  ( 30.00000000000000000, 0.000000000000000000, 0.000000000000000000 ) ) ;
#2297=ORIENTED_EDGE ( 'NONE', *, *, #100, .F. ) ;
#2298=DIRECTION ( 'NONE',  ( 1.000000000000000000, 0.000000000000000000, 0.000000000000000000 ) ) ;
#2299=ORIENTED_EDGE ( 'NONE', *, *, #1638, .F. ) ;
#2303=LINE ( 'NONE', #3157, #131 ) ;
#2308=PLANE ( 'NONE',  #3680 ) ;
#2318=AXIS2_PLACEMENT_3D ( 'NONE', #1660, #3524, #2608 ) ;
#2320=EDGE_CURVE ( 'NONE', #1107, #926, #236, .T. ) ;
#2331=DIRECTION ( 'NONE',  ( -0.000000000000000000, 0.000000000000000000, 1.000000000000000000 ) ) ;
#2337=CARTESIAN_POINT ( 'NONE',  ( -83.12500000000000000, -24.80391854123052653, 5.000000000000000000 ) ) ;
#2345=ORIENTED_EDGE ( 'NONE', *, *, #145, .F. ) ;
#2375=CARTESIAN_POINT ( 'NONE',  ( -80.00000000000000000, 0.000000000000000000, -5.000000000000000000 ) ) ;
#2377=AXIS2_PLACEMENT_3D ( 'NONE', #1560, #3650, #752 ) ;
#2383=ORIENTED_EDGE ( 'NONE', *, *, #2784, .T. ) ;
#2401=EDGE_CURVE ( 'NONE', #1542, #1614, #765, .T. ) ;
#2404=ORIENTED_EDGE ( 'NONE', *, *, #1022, .F. ) ;
#2408=ORIENTED_EDGE ( 'NONE', *, *, #2847, .F. ) ;
#2416=CARTESIAN_POINT ( 'NONE',  ( 30.00000000000000711, 2.696799449851308150, 2.060606060605587597 ) ) ;
#2420=ORIENTED_EDGE ( 'NONE', *, *, #1100, .F. ) ;
#2433=CIRCLE ( 'NONE', #3492, 2.000000000000001776 ) ;
#2442=CIRCLE ( 'NONE', #1763, 2.000000000000001776 ) ;
#2458=ORIENTED_EDGE ( 'NONE', *, *, #1480, .F. ) ;
#2473=CYLINDRICAL_SURFACE ( 'NONE', #1279, 2.000000000000001776 ) ;
#2476=CARTESIAN_POINT ( 'NONE',  ( -82.50000000000000000, -19.84313483298442904, -30.00000000000000000 ) ) ;
#2480=ORIENTED_EDGE ( 'NONE', *, *, #2821, .T. ) ;
#2489=CYLINDRICAL_SURFACE ( 'NONE', #2871, 30.00000000000000000 ) ;
#2506=CARTESIAN_POINT ( 'NONE',  ( 0.000000000000000000, 0.000000000000000000, 0.000000000000000000 ) ) ;
#2507=DIRECTION ( 'NONE',  ( 1.000000000000000000, 0.000000000000000000, 0.000000000000000000 ) ) ;
#2518=FACE_OUTER_BOUND ( 'NONE', #135, .T. ) ;
#2533=DIRECTION ( 'NONE',  ( -0.000000000000000000, 0.000000000000000000, 1.000000000000000000 ) ) ;
#2538=FACE_OUTER_BOUND ( 'NONE', #3569, .T. ) ;
#2542=ORIENTED_EDGE ( 'NONE', *, *, #734, .F. ) ;
#2544=PRODUCT_DEFINITION_CONTEXT ( 'detailed design', #3766, 'design' ) ;
#2547=CARTESIAN_POINT ( 'NONE',  ( -4.374999999999999112, -34.72548595772274638, -30.00000000000000000 ) ) ;
#2557=DIRECTION ( 'NONE',  ( -0.9921567416492214075, 0.1250000000000000555, 0.000000000000000000 ) ) ;
#2560=EDGE_CURVE ( 'NONE', #973, #272, #2442, .T. ) ;
#2579=FACE_BOUND ( 'NONE', #1759, .T. ) ;
#2581=DIRECTION ( 'NONE',  ( -0.000000000000000000, 0.000000000000000000, 1.000000000000000000 ) ) ;
#2584=ADVANCED_FACE ( 'NONE', ( #1050 ), #2167, .T. ) ;
#2587=VERTEX_POINT ( 'NONE', #138 ) ;
#2590=AXIS2_PLACEMENT_3D ( 'NONE', #1128, #1074, #1362 ) ;
#2592=EDGE_CURVE ( 'NONE', #3645, #2149, #2185, .T. ) ;
#2597=VERTEX_POINT ( 'NONE', #3355 ) ;
#2599=CARTESIAN_POINT ( 'NONE',  ( 0.000000000000000000, 0.000000000000000000, 0.000000000000000000 ) ) ;
#2608=DIRECTION ( 'NONE',  ( 1.000000000000000000, 0.000000000000000000, 0.000000000000000000 ) ) ;
#2619=ORIENTED_EDGE ( 'NONE', *, *, #930, .F. ) ;
#2640=DIRECTION ( 'NONE',  ( -0.000000000000000000, 0.000000000000000000, 1.000000000000000000 ) ) ;
#2664=CLOSED_SHELL ( 'NONE', ( #1859, #1866, #3029, #1419, #2939, #250, #2042, #3477, #2098, #860, #845, #3398, #1458, #1042, #3321, #3117, #2584, #3245, #1180, #3278 ) ) ;
#2666=ORIENTED_EDGE ( 'NONE', *, *, #2974, .F. ) ;
#2673=CARTESIAN_POINT ( 'NONE',  ( -83.12500000000000000, -24.80391854123052653, -30.00000000000000000 ) ) ;
#2676=EDGE_LOOP ( 'NONE', ( #2862, #1923, #3466, #2345 ) ) ;
#2691=VECTOR ( 'NONE', #819, 1000.000000000000000 ) ;
#2714=CARTESIAN_POINT ( 'NONE',  ( -89.85223847358115279, -17.40498196091244409, 5.000000000000000000 ) ) ;
#2719=ORIENTED_EDGE ( 'NONE', *, *, #2592, .T. ) ;
#2734=ORIENTED_EDGE ( 'NONE', *, *, #388, .F. ) ;
#2743=DIRECTION ( 'NONE',  ( -1.000000000000000000, 0.000000000000000000, 0.000000000000000000 ) ) ;
#2746=AXIS2_PLACEMENT_3D ( 'NONE', #73, #3022, #2743 ) ;
#2761=AXIS2_PLACEMENT_3D ( 'NONE', #2211, #3400, #735 ) ;
#2774=DIRECTION ( 'NONE',  ( -0.9921567416492215186, 0.1250000000000000833, 0.000000000000000000 ) ) ;
#2784=EDGE_CURVE ( 'NONE', #272, #1614, #356, .T. ) ;
#2793=DIRECTION ( 'NONE',  ( 0.000000000000000000, 1.000000000000000000, 0.000000000000000000 ) ) ;
#2795=CARTESIAN_POINT ( 'NONE',  ( 30.00000000000000000, 0.000000000000000000, -30.00000000000000000 ) ) ;
#2805=CIRCLE ( 'NONE', #3369, 5.000000000000004441 ) ;
#2813=AXIS2_PLACEMENT_3D ( 'NONE', #941, #305, #292 ) ;
#2821=EDGE_CURVE ( 'NONE', #3591, #2597, #1883, .T. ) ;
#2822=AXIS2_PLACEMENT_3D ( 'NONE', #1028, #3068, #2229 ) ;
#2836=ORIENTED_EDGE ( 'NONE', *, *, #382, .T. ) ;
#2840=VERTEX_POINT ( 'NONE', #974 ) ;
#2841=CIRCLE ( 'NONE', #664, 30.00000000000000000 ) ;
#2847=EDGE_CURVE ( 'NONE', #447, #3591, #3264, .T. ) ;
#2850=ORIENTED_EDGE ( 'NONE', *, *, #3281, .T. ) ;
#2851=CARTESIAN_POINT ( 'NONE',  ( -3.750000000000001776, -29.76470224947664178, -30.00000000000000000 ) ) ;
#2852=EDGE_LOOP ( 'NONE', ( #882, #3507, #2542, #571 ) ) ;
#2862=ORIENTED_EDGE ( 'NONE', *, *, #1983, .F. ) ;
#2871=AXIS2_PLACEMENT_3D ( 'NONE', #3675, #3409, #1079 ) ;
#2876=CARTESIAN_POINT ( 'NONE',  ( -82.91666666666667140, -23.15032397181515833, 3.333333333333333037 ) ) ;
#2893=CARTESIAN_POINT ( 'NONE',  ( -82.50000000000000000, -19.84313483298442904, -30.00000000000000000 ) ) ;
#2904=DIRECTION ( 'NONE',  ( 1.000000000000000000, 0.000000000000000000, 0.000000000000000000 ) ) ;
#2912=VERTEX_POINT ( 'NONE', #1900 ) ;
#2927=LINE ( 'NONE', #248, #323 ) ;
#2928=ORIENTED_EDGE ( 'NONE', *, *, #2784, .F. ) ;
#2939=ADVANCED_FACE ( 'NONE', ( #1856 ), #3417, .F. ) ;
#2940=ORIENTED_EDGE ( 'NONE', *, *, #1076, .F. ) ;
#2944=AXIS2_PLACEMENT_3D ( 'NONE', #66, #1468, #3593 ) ;
#2952=EDGE_LOOP ( 'NONE', ( #2299, #651, #1450, #2619 ) ) ;
#2961=CARTESIAN_POINT ( 'NONE',  ( -87.60982564905410186, -19.87129415435180491, 5.000000000000000000 ) ) ;
#2974=EDGE_CURVE ( 'NONE', #2597, #3591, #2014, .T. ) ;
#3018=CARTESIAN_POINT ( 'NONE',  ( -80.00000000000000000, 0.000000000000000000, 0.000000000000000000 ) ) ;
#3022=DIRECTION ( 'NONE',  ( -0.000000000000000000, -0.000000000000000000, -1.000000000000000000 ) ) ;
#3023=( NAMED_UNIT ( * ) SI_UNIT ( $, .STERADIAN. ) SOLID_ANGLE_UNIT ( ) );
#3024=APPLICATION_CONTEXT ( 'automotive_design' ) ;
#3029=ADVANCED_FACE ( 'NONE', ( #222 ), #238, .T. ) ;
#3044=SURFACE_SIDE_STYLE ('',( #3105 ) ) ;
#3049=EDGE_CURVE ( 'NONE', #1107, #910, #1511, .T. ) ;
#3052=VERTEX_POINT ( 'NONE', #1373 ) ;
#3061=CARTESIAN_POINT ( 'NONE',  ( -82.00000000000000000, 0.000000000000000000, -5.000000000000000000 ) ) ;
#3068=DIRECTION ( 'NONE',  ( -0.000000000000000000, -0.000000000000000000, 1.000000000000000000 ) ) ;
#3071=VECTOR ( 'NONE', #1529, 1000.000000000000000 ) ;
#3076=PLANE ( 'NONE',  #704 ) ;
#3086=LINE ( 'NONE', #1574, #832 ) ;
#3099=DIRECTION ( 'NONE',  ( -0.9921567416492215186, 0.1250000000000000833, 0.000000000000000000 ) ) ;
#3105=SURFACE_STYLE_FILL_AREA ( #2198 ) ;
#3114=LINE ( 'NONE', #1860, #1285 ) ;
#3116=ADVANCED_BREP_SHAPE_REPRESENTATION ( '', ( #2021, #2207 ), #3459 ) ;
#3117=ADVANCED_FACE ( 'NONE', ( #2579, #1141 ), #3774, .F. ) ;
#3131=DIRECTION ( 'NONE',  ( 1.000000000000000000, 0.000000000000000000, 0.000000000000000000 ) ) ;
#3142=PLANE ( 'NONE',  #2318 ) ;
#3151=VECTOR ( 'NONE', #1167, 1000.000000000000000 ) ;
#3154=DIRECTION ( 'NONE',  ( 1.000000000000000000, 0.000000000000000000, 0.000000000000000000 ) ) ;
#3157=CARTESIAN_POINT ( 'NONE',  ( -75.00000000000000000, 0.000000000000000000, -5.000000000000000000 ) ) ;
#3161=CYLINDRICAL_SURFACE ( 'NONE', #720, 30.00000000000000000 ) ;
#3171=LINE ( 'NONE', #536, #1221 ) ;
#3172=CARTESIAN_POINT ( 'NONE',  ( 34.99999999999999289, 0.000000000000000000, 4.999999999999997335 ) ) ;
#3174=DIRECTION ( 'NONE',  ( -0.000000000000000000, 0.000000000000000000, 1.000000000000000000 ) ) ;
#3180=ORIENTED_EDGE ( 'NONE', *, *, #3649, .F. ) ;
#3193=CARTESIAN_POINT ( 'NONE',  ( 0.000000000000000000, 0.000000000000000000, -30.00000000000000000 ) ) ;
#3194=DIRECTION ( 'NONE',  ( 1.000000000000000000, 0.000000000000000000, 0.000000000000000000 ) ) ;
#3199=EDGE_LOOP ( 'NONE', ( #709, #2212, #3413 ) ) ;
#3206=VECTOR ( 'NONE', #2160, 1000.000000000000000 ) ;
#3221=ORIENTED_EDGE ( 'NONE', *, *, #382, .F. ) ;
#3222=CARTESIAN_POINT ( 'NONE',  ( -80.00000000000000000, 0.000000000000000000, 0.000000000000000000 ) ) ;
#3242=CIRCLE ( 'NONE', #1384, 34.99999999999999289 ) ;
#3245=ADVANCED_FACE ( 'NONE', ( #965, #407 ), #329, .T. ) ;
#3256=ORIENTED_EDGE ( 'NONE', *, *, #2592, .F. ) ;
#3264=LINE ( 'NONE', #3345, #3687 ) ;
#3274=CARTESIAN_POINT ( 'NONE',  ( -4.374999999999999112, -34.72548595772274638, 4.999999999999997335 ) ) ;
#3275=ORIENTED_EDGE ( 'NONE', *, *, #1052, .F. ) ;
#3278=ADVANCED_FACE ( 'NONE', ( #2518 ), #2148, .F. ) ;
#3281=EDGE_CURVE ( 'NONE', #2012, #821, #3353, .T. ) ;
#3307=AXIS2_PLACEMENT_3D ( 'NONE', #743, #1924, #1343 ) ;
#3316=ORIENTED_EDGE ( 'NONE', *, *, #157, .F. ) ;
#3321=ADVANCED_FACE ( 'NONE', ( #194 ), #3769, .T. ) ;
#3322=ORIENTED_EDGE ( 'NONE', *, *, #422, .T. ) ;
#3324=CARTESIAN_POINT ( 'NONE',  ( -78.00000000000000000, 2.449293598294708880E-16, -5.000000000000000000 ) ) ;
#3334=PRODUCT_DEFINITION_FORMATION_WITH_SPECIFIED_SOURCE ( 'ANY', '', #343, .NOT_KNOWN. ) ;
#3339=DIRECTION ( 'NONE',  ( 0.000000000000000000, 0.000000000000000000, 1.000000000000000000 ) ) ;
#3345=CARTESIAN_POINT ( 'NONE',  ( -85.00000000000000000, 6.123233995736771213E-16, -5.000000000000000000 ) ) ;
#3348=CARTESIAN_POINT ( 'NONE',  ( -83.12500000000000000, -24.80391854123052653, -30.00000000000000000 ) ) ;
#3353=LINE ( 'NONE', #2476, #1567 ) ;
#3354=ORIENTED_EDGE ( 'NONE', *, *, #1657, .F. ) ;
#3355=CARTESIAN_POINT ( 'NONE',  ( -75.00000000000000000, 0.000000000000000000, 0.000000000000000000 ) ) ;
#3363=DIRECTION ( 'NONE',  ( 0.000000000000000000, 0.000000000000000000, 1.000000000000000000 ) ) ;
#3365=( NAMED_UNIT ( * ) PLANE_ANGLE_UNIT ( ) SI_UNIT ( $, .RADIAN. ) );
#3369=AXIS2_PLACEMENT_3D ( 'NONE', #2375, #3837, #3783 ) ;
#3386=ORIENTED_EDGE ( 'NONE', *, *, #2102, .T. ) ;
#3387=DIRECTION ( 'NONE',  ( -0.000000000000000000, 0.000000000000000000, 1.000000000000000000 ) ) ;
#3394=EDGE_LOOP ( 'NONE', ( #2458, #773, #2480, #2297 ) ) ;
#3398=ADVANCED_FACE ( 'NONE', ( #1106 ), #2308, .F. ) ;
#3400=DIRECTION ( 'NONE',  ( 0.000000000000000000, -0.000000000000000000, -1.000000000000000000 ) ) ;
#3401=ORIENTED_EDGE ( 'NONE', *, *, #1066, .T. ) ;
#3407=CYLINDRICAL_SURFACE ( 'NONE', #3307, 2.000000000000001776 ) ;
#3409=DIRECTION ( 'NONE',  ( -0.000000000000000000, 0.000000000000000000, 1.000000000000000000 ) ) ;
#3413=ORIENTED_EDGE ( 'NONE', *, *, #1939, .T. ) ;
#3416=EDGE_CURVE ( 'NONE', #2149, #3455, #1725, .T. ) ;
#3417=PLANE ( 'NONE',  #2377 ) ;
#3419=CARTESIAN_POINT ( 'NONE',  ( -78.00000000000000000, 2.449293598294708880E-16, 3.000000000000000000 ) ) ;
#3438=DIRECTION ( 'NONE',  ( 0.000000000000000000, 0.000000000000000000, 1.000000000000000000 ) ) ;
#3449=EDGE_CURVE ( 'NONE', #1755, #910, #490, .T. ) ;
#3452=VECTOR ( 'NONE', #951, 1000.000000000000000 ) ;
#3454=AXIS2_PLACEMENT_3D ( 'NONE', #392, #2793, #3733 ) ;
#3455=VERTEX_POINT ( 'NONE', #2714 ) ;
#3456=CARTESIAN_POINT ( 'NONE',  ( -83.83626752599590759, -19.67478094923029985, 1.151994720958518181 ) ) ;
#3459=( GEOMETRIC_REPRESENTATION_CONTEXT ( 3 ) GLOBAL_UNCERTAINTY_ASSIGNED_CONTEXT ( ( #828 ) ) GLOBAL_UNIT_ASSIGNED_CONTEXT ( ( #45, #3365, #3023 ) ) REPRESENTATION_CONTEXT ( 'NONE', 'WORKASPACE' ) );
#3460=CIRCLE ( 'NONE', #913, 30.00000000000000000 ) ;
#3465=CARTESIAN_POINT ( 'NONE',  ( 31.66666666666666075, 0.000000000000000000, 1.666666666666665630 ) ) ;
#3466=ORIENTED_EDGE ( 'NONE', *, *, #3416, .T. ) ;
#3470=CARTESIAN_POINT ( 'NONE',  ( -4.375000000000001776, -34.72548595772274638, -30.00000000000000000 ) ) ;
#3477=ADVANCED_FACE ( 'NONE', ( #1796 ), #47, .T. ) ;
#3484=CARTESIAN_POINT ( 'NONE',  ( -3.750000000000004441, 29.76470224947664533, 0.000000000000000000 ) ) ;
#3489=VERTEX_POINT ( 'NONE', #3274 ) ;
#3492=AXIS2_PLACEMENT_3D ( 'NONE', #3602, #1512, #1231 ) ;
#3507=ORIENTED_EDGE ( 'NONE', *, *, #2320, .T. ) ;
#3515=( GEOMETRIC_REPRESENTATION_CONTEXT ( 3 ) GLOBAL_UNCERTAINTY_ASSIGNED_CONTEXT ( ( #1643 ) ) GLOBAL_UNIT_ASSIGNED_CONTEXT ( ( #680, #2162, #663 ) ) REPRESENTATION_CONTEXT ( 'NONE', 'WORKASPACE' ) );
#3524=DIRECTION ( 'NONE',  ( -0.000000000000000000, 0.000000000000000000, 1.000000000000000000 ) ) ;
#3531=LINE ( 'NONE', #1179, #403 ) ;
#3554=CARTESIAN_POINT ( 'NONE',  ( -82.50000000000000000, -19.84313483298442904, -30.00000000000000000 ) ) ;
#3569=EDGE_LOOP ( 'NONE', ( #86, #2836, #1157, #3180 ) ) ;
#3591=VERTEX_POINT ( 'NONE', #27 ) ;
#3593=DIRECTION ( 'NONE',  ( -1.000000000000000000, 0.000000000000000000, 0.000000000000000000 ) ) ;
#3594=EDGE_CURVE ( 'NONE', #3489, #2587, #2927, .T. ) ;
#3596=DIRECTION ( 'NONE',  ( 0.000000000000000000, -0.000000000000000000, -1.000000000000000000 ) ) ;
#3597=DIRECTION ( 'NONE',  ( -0.000000000000000000, 0.000000000000000000, 1.000000000000000000 ) ) ;
#3602=CARTESIAN_POINT ( 'NONE',  ( -80.00000000000000000, 0.000000000000000000, 3.000000000000000000 ) ) ;
#3610=ORIENTED_EDGE ( 'NONE', *, *, #1849, .F. ) ;
#3637=AXIS2_PLACEMENT_3D ( 'NONE', #1313, #119, #3131 ) ;
#3641=CARTESIAN_POINT ( 'NONE',  ( -80.00000000000000000, 0.000000000000000000, -5.000000000000000000 ) ) ;
#3645=VERTEX_POINT ( 'NONE', #706 ) ;
#3649=EDGE_CURVE ( 'NONE', #2084, #1107, #3086, .T. ) ;
#3650=DIRECTION ( 'NONE',  ( 0.1250000000000001665, -0.9921567416492215186, 0.000000000000000000 ) ) ;
#3651=EDGE_LOOP ( 'NONE', ( #2734, #753, #2383, #613 ) ) ;
#3654=DIRECTION ( 'NONE',  ( 0.3736424900038657904, -0.8444627602987255788, 0.3837628644519533450 ) ) ;
#3661=ORIENTED_EDGE ( 'NONE', *, *, #100, .T. ) ;
#3670=FACE_OUTER_BOUND ( 'NONE', #506, .T. ) ;
#3675=CARTESIAN_POINT ( 'NONE',  ( 0.000000000000000000, 0.000000000000000000, 0.000000000000000000 ) ) ;
#3680=AXIS2_PLACEMENT_3D ( 'NONE', #3470, #2271, #806 ) ;
#3687=VECTOR ( 'NONE', #2156, 1000.000000000000000 ) ;
#3689=ORIENTED_EDGE ( 'NONE', *, *, #151, .T. ) ;
#3696=DIRECTION ( 'NONE',  ( 1.000000000000000000, 0.000000000000000000, 0.000000000000000000 ) ) ;
#3706=CIRCLE ( 'NONE', #1584, 20.00000000000000355 ) ;
#3708=DIRECTION ( 'NONE',  ( 0.000000000000000000, 0.000000000000000000, -1.000000000000000000 ) ) ;
#3713=ORIENTED_EDGE ( 'NONE', *, *, #422, .F. ) ;
#3733=DIRECTION ( 'NONE',  ( 0.000000000000000000, 0.000000000000000000, 1.000000000000000000 ) ) ;
#3753=DIRECTION ( 'NONE',  ( 1.000000000000000000, 0.000000000000000000, 0.000000000000000000 ) ) ;
#3758=LINE ( 'NONE', #1038, #822 ) ;
#3766=APPLICATION_CONTEXT ( 'automotive_design' ) ;
#3769=PLANE ( 'NONE',  #1756 ) ;
#3774=PLANE ( 'NONE',  #327 ) ;
#3782=EDGE_CURVE ( 'NONE', #926, #1166, #269, .T. ) ;
#3783=DIRECTION ( 'NONE',  ( -1.000000000000000000, 0.000000000000000000, 0.000000000000000000 ) ) ;
#3784=CARTESIAN_POINT ( 'NONE',  ( 30.95238095238181231, 5.297284633636610174, 5.000000000000000000 ) ) ;
#3786=CARTESIAN_POINT ( 'NONE',  ( -88.76305748969319609, -18.02152214568556943, 4.485328054291851885 ) ) ;
#3833=CARTESIAN_POINT ( 'NONE',  ( -89.85223847358115279, -17.40498196091244409, 5.000000000000000000 ) ) ;
#3837=DIRECTION ( 'NONE',  ( 0.000000000000000000, 0.000000000000000000, -1.000000000000000000 ) ) ;
#3854=COLOUR_RGB('Light Blue',0.38,0.62,0.78);
#3855=FILL_AREA_STYLE_COLOUR('',#3854);
#3856=FILL_AREA_STYLE('',(#3855));
#3857=SURFACE_STYLE_FILL_AREA(#3856);
#3858=SURFACE_SIDE_STYLE('',(#3857));
#3859=SURFACE_STYLE_USAGE(.BOTH.,#3858);
#3860=PRESENTATION_STYLE_ASSIGNMENT((#3859));
ENDSEC;
END-ISO-10303-21;
